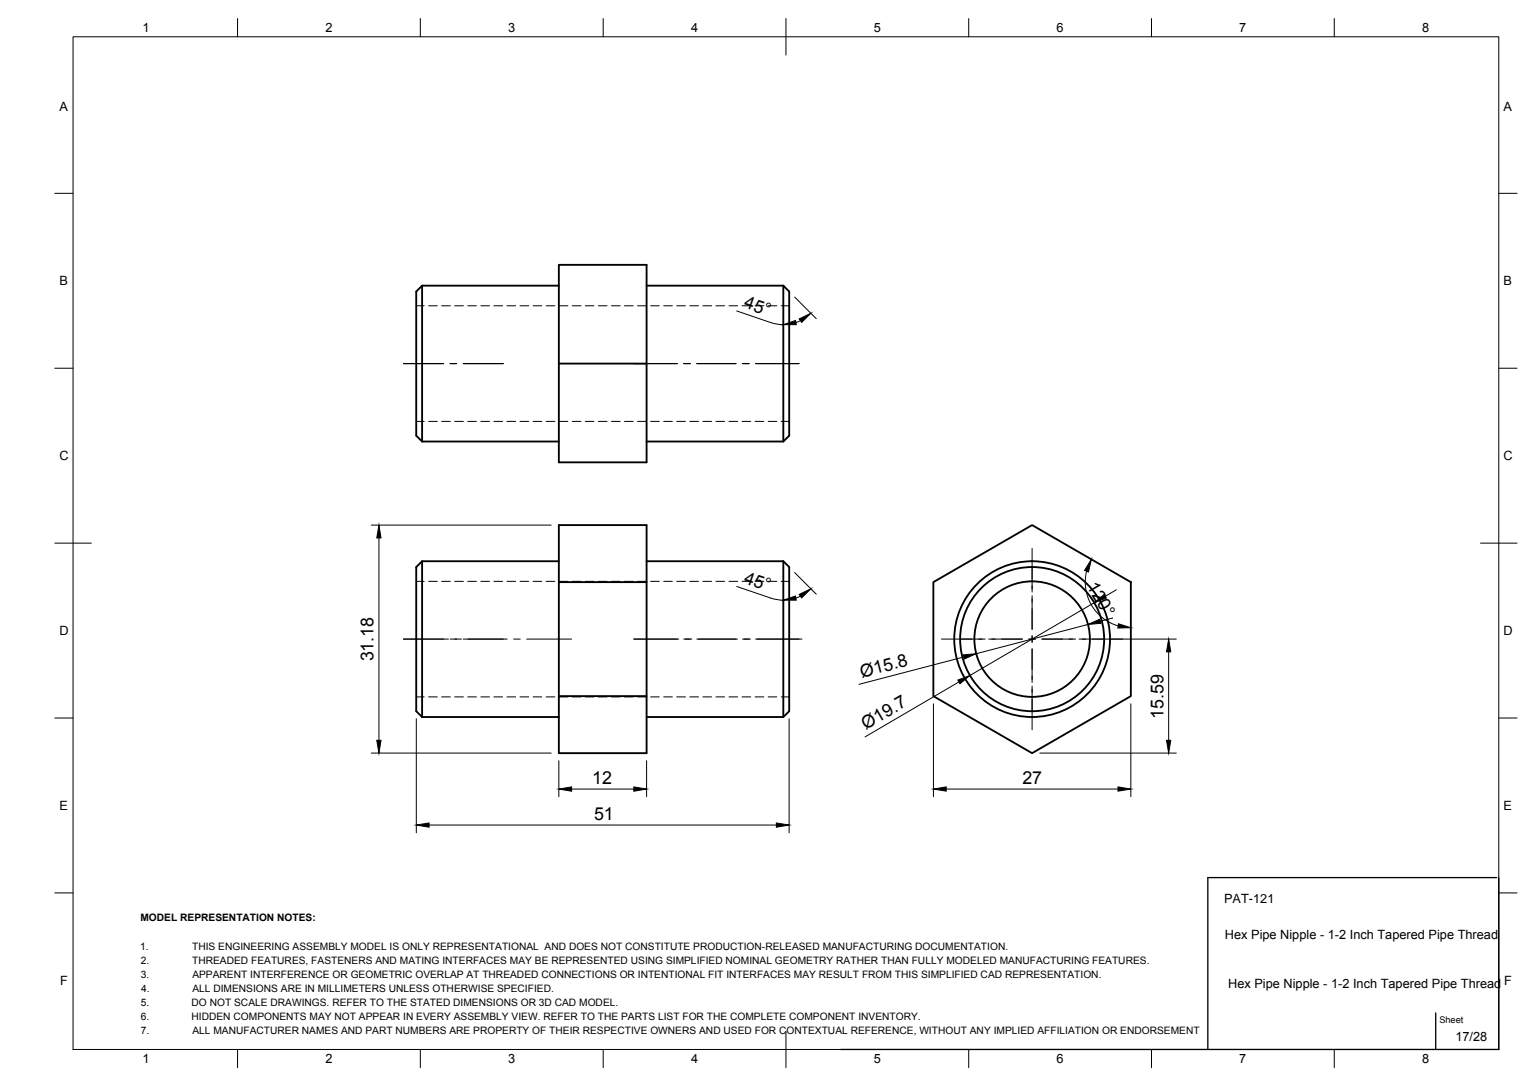
ISO-10303-21;
HEADER;
/* Generated by software containing ST-Developer
 * from STEP Tools, Inc. (www.steptools.com) 
 */

FILE_DESCRIPTION(
/* description */ ('Wall-mounted air drop station'),
/* implementation_level */ '2;1');

FILE_NAME(
/* name */ 'Hex Pipe Nipple - 1-2 Inch Tapered Pipe Thread.step',
/* time_stamp */ '2026-10-28T22:16:19-07:00',
/* author */ (''),
/* organization */ (''),
/* preprocessor_version */ 'ST-DEVELOPER v20.2',
/* originating_system */ 'Autodesk Translation Framework v15.17.0.0',
/* authorisation */ '');

FILE_SCHEMA (('AUTOMOTIVE_DESIGN { 1 0 10303 214 3 1 1 }'));
ENDSEC;

DATA;
#10=MECHANICAL_DESIGN_GEOMETRIC_PRESENTATION_REPRESENTATION('',(#360),#10517);
#273=CONICAL_SURFACE('',#6636,1.025,0.785398163397448);
#274=CONICAL_SURFACE('',#6639,1.025,0.785398163397448);
#302=SHAPE_REPRESENTATION_RELATIONSHIP('SRR','None',#10659,#331);
#331=ADVANCED_BREP_SHAPE_REPRESENTATION('',(#388),#10503);
#360=STYLED_ITEM('',(#10860),#388);
#388=MANIFOLD_SOLID_BREP('Body1',#5900);
#498=FACE_BOUND('',#1418,.T.);
#499=FACE_BOUND('',#1420,.T.);
#500=FACE_BOUND('',#1429,.T.);
#501=FACE_BOUND('',#1434,.T.);
#651=PLANE('',#6621);
#652=PLANE('',#6623);
#653=PLANE('',#6625);
#654=PLANE('',#6626);
#655=PLANE('',#6627);
#656=PLANE('',#6628);
#657=PLANE('',#6629);
#658=PLANE('',#6630);
#659=PLANE('',#6633);
#660=PLANE('',#6641);
#963=FACE_OUTER_BOUND('',#1417,.T.);
#964=FACE_OUTER_BOUND('',#1419,.T.);
#965=FACE_OUTER_BOUND('',#1421,.T.);
#966=FACE_OUTER_BOUND('',#1422,.T.);
#967=FACE_OUTER_BOUND('',#1423,.T.);
#968=FACE_OUTER_BOUND('',#1424,.T.);
#969=FACE_OUTER_BOUND('',#1425,.T.);
#970=FACE_OUTER_BOUND('',#1426,.T.);
#971=FACE_OUTER_BOUND('',#1427,.T.);
#972=FACE_OUTER_BOUND('',#1428,.T.);
#973=FACE_OUTER_BOUND('',#1430,.T.);
#974=FACE_OUTER_BOUND('',#1431,.T.);
#975=FACE_OUTER_BOUND('',#1432,.T.);
#976=FACE_OUTER_BOUND('',#1433,.T.);
#977=FACE_OUTER_BOUND('',#1435,.T.);
#1417=EDGE_LOOP('',(#4843,#4844,#4845,#4846,#4847,#4848));
#1418=EDGE_LOOP('',(#4849));
#1419=EDGE_LOOP('',(#4850,#4851,#4852,#4853,#4854,#4855));
#1420=EDGE_LOOP('',(#4856));
#1421=EDGE_LOOP('',(#4857,#4858,#4859,#4860));
#1422=EDGE_LOOP('',(#4861,#4862,#4863,#4864));
#1423=EDGE_LOOP('',(#4865,#4866,#4867,#4868));
#1424=EDGE_LOOP('',(#4869,#4870,#4871,#4872));
#1425=EDGE_LOOP('',(#4873,#4874,#4875,#4876));
#1426=EDGE_LOOP('',(#4877,#4878,#4879,#4880));
#1427=EDGE_LOOP('',(#4881,#4882,#4883,#4884));
#1428=EDGE_LOOP('',(#4885));
#1429=EDGE_LOOP('',(#4886));
#1430=EDGE_LOOP('',(#4887,#4888,#4889,#4890));
#1431=EDGE_LOOP('',(#4891,#4892,#4893,#4894));
#1432=EDGE_LOOP('',(#4895,#4896,#4897,#4898));
#1433=EDGE_LOOP('',(#4899));
#1434=EDGE_LOOP('',(#4900));
#1435=EDGE_LOOP('',(#4901,#4902,#4903,#4904));
#1856=LINE('',#9743,#2320);
#1857=LINE('',#9745,#2321);
#1858=LINE('',#9747,#2322);
#1859=LINE('',#9749,#2323);
#1860=LINE('',#9751,#2324);
#1861=LINE('',#9752,#2325);
#1862=LINE('',#9758,#2326);
#1863=LINE('',#9760,#2327);
#1864=LINE('',#9762,#2328);
#1865=LINE('',#9764,#2329);
#1866=LINE('',#9766,#2330);
#1867=LINE('',#9767,#2331);
#1868=LINE('',#9771,#2332);
#1869=LINE('',#9772,#2333);
#1870=LINE('',#9774,#2334);
#1871=LINE('',#9776,#2335);
#1872=LINE('',#9778,#2336);
#1873=LINE('',#9780,#2337);
#1874=LINE('',#9784,#2338);
#1875=LINE('',#9792,#2339);
#1876=LINE('',#9796,#2340);
#1877=LINE('',#9800,#2341);
#1878=LINE('',#9805,#2342);
#2320=VECTOR('',#7962,1.);
#2321=VECTOR('',#7963,1.);
#2322=VECTOR('',#7964,1.);
#2323=VECTOR('',#7965,1.);
#2324=VECTOR('',#7966,1.);
#2325=VECTOR('',#7967,1.);
#2326=VECTOR('',#7972,1.);
#2327=VECTOR('',#7973,1.);
#2328=VECTOR('',#7974,1.);
#2329=VECTOR('',#7975,1.);
#2330=VECTOR('',#7976,1.);
#2331=VECTOR('',#7977,1.);
#2332=VECTOR('',#7982,1.);
#2333=VECTOR('',#7983,1.);
#2334=VECTOR('',#7986,1.);
#2335=VECTOR('',#7989,1.);
#2336=VECTOR('',#7992,1.);
#2337=VECTOR('',#7995,1.);
#2338=VECTOR('',#8000,1.065);
#2339=VECTOR('',#8011,1.025);
#2340=VECTOR('',#8016,1.065);
#2341=VECTOR('',#8021,1.025);
#2342=VECTOR('',#8028,0.79);
#2679=CIRCLE('',#6622,1.065);
#2680=CIRCLE('',#6624,1.065);
#2681=CIRCLE('',#6632,1.065);
#2682=CIRCLE('',#6634,0.985);
#2683=CIRCLE('',#6635,0.79);
#2684=CIRCLE('',#6638,1.065);
#2685=CIRCLE('',#6640,0.985);
#2686=CIRCLE('',#6642,0.79);
#3053=VERTEX_POINT('',#9741);
#3054=VERTEX_POINT('',#9742);
#3055=VERTEX_POINT('',#9744);
#3056=VERTEX_POINT('',#9746);
#3057=VERTEX_POINT('',#9748);
#3058=VERTEX_POINT('',#9750);
#3059=VERTEX_POINT('',#9753);
#3060=VERTEX_POINT('',#9756);
#3061=VERTEX_POINT('',#9757);
#3062=VERTEX_POINT('',#9759);
#3063=VERTEX_POINT('',#9761);
#3064=VERTEX_POINT('',#9763);
#3065=VERTEX_POINT('',#9765);
#3066=VERTEX_POINT('',#9768);
#3067=VERTEX_POINT('',#9783);
#3068=VERTEX_POINT('',#9787);
#3069=VERTEX_POINT('',#9789);
#3070=VERTEX_POINT('',#9794);
#3071=VERTEX_POINT('',#9798);
#3072=VERTEX_POINT('',#9802);
#3679=EDGE_CURVE('',#3053,#3054,#1856,.T.);
#3680=EDGE_CURVE('',#3054,#3055,#1857,.T.);
#3681=EDGE_CURVE('',#3055,#3056,#1858,.T.);
#3682=EDGE_CURVE('',#3056,#3057,#1859,.T.);
#3683=EDGE_CURVE('',#3057,#3058,#1860,.T.);
#3684=EDGE_CURVE('',#3058,#3053,#1861,.T.);
#3685=EDGE_CURVE('',#3059,#3059,#2679,.T.);
#3686=EDGE_CURVE('',#3060,#3061,#1862,.T.);
#3687=EDGE_CURVE('',#3061,#3062,#1863,.T.);
#3688=EDGE_CURVE('',#3062,#3063,#1864,.T.);
#3689=EDGE_CURVE('',#3063,#3064,#1865,.T.);
#3690=EDGE_CURVE('',#3064,#3065,#1866,.T.);
#3691=EDGE_CURVE('',#3065,#3060,#1867,.T.);
#3692=EDGE_CURVE('',#3066,#3066,#2680,.T.);
#3693=EDGE_CURVE('',#3060,#3054,#1868,.T.);
#3694=EDGE_CURVE('',#3055,#3065,#1869,.T.);
#3695=EDGE_CURVE('',#3056,#3064,#1870,.T.);
#3696=EDGE_CURVE('',#3057,#3063,#1871,.T.);
#3697=EDGE_CURVE('',#3058,#3062,#1872,.T.);
#3698=EDGE_CURVE('',#3053,#3061,#1873,.T.);
#3699=EDGE_CURVE('',#3066,#3067,#1874,.T.);
#3700=EDGE_CURVE('',#3067,#3067,#2681,.T.);
#3701=EDGE_CURVE('',#3068,#3068,#2682,.T.);
#3702=EDGE_CURVE('',#3069,#3069,#2683,.T.);
#3703=EDGE_CURVE('',#3067,#3068,#1875,.T.);
#3704=EDGE_CURVE('',#3070,#3070,#2684,.T.);
#3705=EDGE_CURVE('',#3070,#3059,#1876,.T.);
#3706=EDGE_CURVE('',#3071,#3071,#2685,.T.);
#3707=EDGE_CURVE('',#3071,#3070,#1877,.T.);
#3708=EDGE_CURVE('',#3072,#3072,#2686,.T.);
#3709=EDGE_CURVE('',#3072,#3069,#1878,.T.);
#4843=ORIENTED_EDGE('',*,*,#3679,.T.);
#4844=ORIENTED_EDGE('',*,*,#3680,.T.);
#4845=ORIENTED_EDGE('',*,*,#3681,.T.);
#4846=ORIENTED_EDGE('',*,*,#3682,.T.);
#4847=ORIENTED_EDGE('',*,*,#3683,.T.);
#4848=ORIENTED_EDGE('',*,*,#3684,.T.);
#4849=ORIENTED_EDGE('',*,*,#3685,.F.);
#4850=ORIENTED_EDGE('',*,*,#3686,.T.);
#4851=ORIENTED_EDGE('',*,*,#3687,.T.);
#4852=ORIENTED_EDGE('',*,*,#3688,.T.);
#4853=ORIENTED_EDGE('',*,*,#3689,.T.);
#4854=ORIENTED_EDGE('',*,*,#3690,.T.);
#4855=ORIENTED_EDGE('',*,*,#3691,.T.);
#4856=ORIENTED_EDGE('',*,*,#3692,.F.);
#4857=ORIENTED_EDGE('',*,*,#3693,.F.);
#4858=ORIENTED_EDGE('',*,*,#3691,.F.);
#4859=ORIENTED_EDGE('',*,*,#3694,.F.);
#4860=ORIENTED_EDGE('',*,*,#3680,.F.);
#4861=ORIENTED_EDGE('',*,*,#3694,.T.);
#4862=ORIENTED_EDGE('',*,*,#3690,.F.);
#4863=ORIENTED_EDGE('',*,*,#3695,.F.);
#4864=ORIENTED_EDGE('',*,*,#3681,.F.);
#4865=ORIENTED_EDGE('',*,*,#3695,.T.);
#4866=ORIENTED_EDGE('',*,*,#3689,.F.);
#4867=ORIENTED_EDGE('',*,*,#3696,.F.);
#4868=ORIENTED_EDGE('',*,*,#3682,.F.);
#4869=ORIENTED_EDGE('',*,*,#3696,.T.);
#4870=ORIENTED_EDGE('',*,*,#3688,.F.);
#4871=ORIENTED_EDGE('',*,*,#3697,.F.);
#4872=ORIENTED_EDGE('',*,*,#3683,.F.);
#4873=ORIENTED_EDGE('',*,*,#3697,.T.);
#4874=ORIENTED_EDGE('',*,*,#3687,.F.);
#4875=ORIENTED_EDGE('',*,*,#3698,.F.);
#4876=ORIENTED_EDGE('',*,*,#3684,.F.);
#4877=ORIENTED_EDGE('',*,*,#3698,.T.);
#4878=ORIENTED_EDGE('',*,*,#3686,.F.);
#4879=ORIENTED_EDGE('',*,*,#3693,.T.);
#4880=ORIENTED_EDGE('',*,*,#3679,.F.);
#4881=ORIENTED_EDGE('',*,*,#3692,.T.);
#4882=ORIENTED_EDGE('',*,*,#3699,.T.);
#4883=ORIENTED_EDGE('',*,*,#3700,.T.);
#4884=ORIENTED_EDGE('',*,*,#3699,.F.);
#4885=ORIENTED_EDGE('',*,*,#3701,.F.);
#4886=ORIENTED_EDGE('',*,*,#3702,.T.);
#4887=ORIENTED_EDGE('',*,*,#3700,.F.);
#4888=ORIENTED_EDGE('',*,*,#3703,.T.);
#4889=ORIENTED_EDGE('',*,*,#3701,.T.);
#4890=ORIENTED_EDGE('',*,*,#3703,.F.);
#4891=ORIENTED_EDGE('',*,*,#3704,.F.);
#4892=ORIENTED_EDGE('',*,*,#3705,.T.);
#4893=ORIENTED_EDGE('',*,*,#3685,.T.);
#4894=ORIENTED_EDGE('',*,*,#3705,.F.);
#4895=ORIENTED_EDGE('',*,*,#3706,.F.);
#4896=ORIENTED_EDGE('',*,*,#3707,.T.);
#4897=ORIENTED_EDGE('',*,*,#3704,.T.);
#4898=ORIENTED_EDGE('',*,*,#3707,.F.);
#4899=ORIENTED_EDGE('',*,*,#3706,.T.);
#4900=ORIENTED_EDGE('',*,*,#3708,.F.);
#4901=ORIENTED_EDGE('',*,*,#3708,.T.);
#4902=ORIENTED_EDGE('',*,*,#3709,.T.);
#4903=ORIENTED_EDGE('',*,*,#3702,.F.);
#4904=ORIENTED_EDGE('',*,*,#3709,.F.);
#5501=CYLINDRICAL_SURFACE('',#6631,1.065);
#5502=CYLINDRICAL_SURFACE('',#6637,1.065);
#5503=CYLINDRICAL_SURFACE('',#6643,0.79);
#5736=ADVANCED_FACE('',(#963,#498),#651,.F.);
#5737=ADVANCED_FACE('',(#964,#499),#652,.T.);
#5738=ADVANCED_FACE('',(#965),#653,.T.);
#5739=ADVANCED_FACE('',(#966),#654,.T.);
#5740=ADVANCED_FACE('',(#967),#655,.T.);
#5741=ADVANCED_FACE('',(#968),#656,.T.);
#5742=ADVANCED_FACE('',(#969),#657,.T.);
#5743=ADVANCED_FACE('',(#970),#658,.T.);
#5744=ADVANCED_FACE('',(#971),#5501,.T.);
#5745=ADVANCED_FACE('',(#972,#500),#659,.T.);
#5746=ADVANCED_FACE('',(#973),#273,.T.);
#5747=ADVANCED_FACE('',(#974),#5502,.T.);
#5748=ADVANCED_FACE('',(#975),#274,.T.);
#5749=ADVANCED_FACE('',(#976,#501),#660,.T.);
#5750=ADVANCED_FACE('',(#977),#5503,.F.);
#5900=CLOSED_SHELL('',(#5736,#5737,#5738,#5739,#5740,#5741,#5742,#5743,
#5744,#5745,#5746,#5747,#5748,#5749,#5750));
#6620=AXIS2_PLACEMENT_3D('',#9739,#7958,#7959);
#6621=AXIS2_PLACEMENT_3D('',#9740,#7960,#7961);
#6622=AXIS2_PLACEMENT_3D('',#9754,#7968,#7969);
#6623=AXIS2_PLACEMENT_3D('',#9755,#7970,#7971);
#6624=AXIS2_PLACEMENT_3D('',#9769,#7978,#7979);
#6625=AXIS2_PLACEMENT_3D('',#9770,#7980,#7981);
#6626=AXIS2_PLACEMENT_3D('',#9773,#7984,#7985);
#6627=AXIS2_PLACEMENT_3D('',#9775,#7987,#7988);
#6628=AXIS2_PLACEMENT_3D('',#9777,#7990,#7991);
#6629=AXIS2_PLACEMENT_3D('',#9779,#7993,#7994);
#6630=AXIS2_PLACEMENT_3D('',#9781,#7996,#7997);
#6631=AXIS2_PLACEMENT_3D('',#9782,#7998,#7999);
#6632=AXIS2_PLACEMENT_3D('',#9785,#8001,#8002);
#6633=AXIS2_PLACEMENT_3D('',#9786,#8003,#8004);
#6634=AXIS2_PLACEMENT_3D('',#9788,#8005,#8006);
#6635=AXIS2_PLACEMENT_3D('',#9790,#8007,#8008);
#6636=AXIS2_PLACEMENT_3D('',#9791,#8009,#8010);
#6637=AXIS2_PLACEMENT_3D('',#9793,#8012,#8013);
#6638=AXIS2_PLACEMENT_3D('',#9795,#8014,#8015);
#6639=AXIS2_PLACEMENT_3D('',#9797,#8017,#8018);
#6640=AXIS2_PLACEMENT_3D('',#9799,#8019,#8020);
#6641=AXIS2_PLACEMENT_3D('',#9801,#8022,#8023);
#6642=AXIS2_PLACEMENT_3D('',#9803,#8024,#8025);
#6643=AXIS2_PLACEMENT_3D('',#9804,#8026,#8027);
#7958=DIRECTION('axis',(0.,0.,1.));
#7959=DIRECTION('refdir',(1.,0.,0.));
#7960=DIRECTION('center_axis',(0.,1.,0.));
#7961=DIRECTION('ref_axis',(1.,0.,0.));
#7962=DIRECTION('',(-0.5,0.,0.866025403784439));
#7963=DIRECTION('',(-1.,0.,-2.84883360945713E-16));
#7964=DIRECTION('',(-0.5,0.,-0.866025403784439));
#7965=DIRECTION('',(0.5,0.,-0.866025403784439));
#7966=DIRECTION('',(1.,0.,0.));
#7967=DIRECTION('',(0.5,0.,0.866025403784439));
#7968=DIRECTION('center_axis',(0.,-1.,0.));
#7969=DIRECTION('ref_axis',(1.,0.,0.));
#7970=DIRECTION('center_axis',(0.,1.,0.));
#7971=DIRECTION('ref_axis',(1.,0.,0.));
#7972=DIRECTION('',(0.5,0.,-0.866025403784439));
#7973=DIRECTION('',(-0.5,0.,-0.866025403784439));
#7974=DIRECTION('',(-1.,0.,0.));
#7975=DIRECTION('',(-0.5,0.,0.866025403784439));
#7976=DIRECTION('',(0.5,0.,0.866025403784439));
#7977=DIRECTION('',(1.,0.,2.84883360945713E-16));
#7978=DIRECTION('center_axis',(0.,1.,0.));
#7979=DIRECTION('ref_axis',(1.,0.,0.));
#7980=DIRECTION('center_axis',(-2.84883360945713E-16,0.,1.));
#7981=DIRECTION('ref_axis',(1.,0.,2.84883360945713E-16));
#7982=DIRECTION('',(0.,-1.,0.));
#7983=DIRECTION('',(0.,1.,0.));
#7984=DIRECTION('center_axis',(-0.866025403784439,0.,0.5));
#7985=DIRECTION('ref_axis',(0.5,0.,0.866025403784439));
#7986=DIRECTION('',(0.,1.,0.));
#7987=DIRECTION('center_axis',(-0.866025403784439,0.,-0.5));
#7988=DIRECTION('ref_axis',(-0.5,0.,0.866025403784439));
#7989=DIRECTION('',(0.,1.,0.));
#7990=DIRECTION('center_axis',(0.,0.,-1.));
#7991=DIRECTION('ref_axis',(-1.,0.,0.));
#7992=DIRECTION('',(0.,1.,0.));
#7993=DIRECTION('center_axis',(0.866025403784439,0.,-0.5));
#7994=DIRECTION('ref_axis',(-0.5,0.,-0.866025403784439));
#7995=DIRECTION('',(0.,1.,0.));
#7996=DIRECTION('center_axis',(0.866025403784439,0.,0.5));
#7997=DIRECTION('ref_axis',(0.5,0.,-0.866025403784439));
#7998=DIRECTION('center_axis',(0.,-1.,0.));
#7999=DIRECTION('ref_axis',(1.,0.,0.));
#8000=DIRECTION('',(0.,1.,0.));
#8001=DIRECTION('center_axis',(0.,-1.,0.));
#8002=DIRECTION('ref_axis',(1.,0.,0.));
#8003=DIRECTION('center_axis',(0.,1.,0.));
#8004=DIRECTION('ref_axis',(0.,0.,1.));
#8005=DIRECTION('center_axis',(0.,-1.,0.));
#8006=DIRECTION('ref_axis',(1.,0.,0.));
#8007=DIRECTION('center_axis',(0.,-1.,0.));
#8008=DIRECTION('ref_axis',(1.,0.,0.));
#8009=DIRECTION('center_axis',(0.,-1.,0.));
#8010=DIRECTION('ref_axis',(1.,0.,0.));
#8011=DIRECTION('',(0.707106781186547,0.707106781186548,8.65956056235493E-17));
#8012=DIRECTION('center_axis',(0.,-1.,0.));
#8013=DIRECTION('ref_axis',(1.,0.,0.));
#8014=DIRECTION('center_axis',(0.,-1.,0.));
#8015=DIRECTION('ref_axis',(1.,0.,0.));
#8016=DIRECTION('',(0.,1.,0.));
#8017=DIRECTION('center_axis',(0.,1.,0.));
#8018=DIRECTION('ref_axis',(1.,0.,0.));
#8019=DIRECTION('center_axis',(0.,-1.,0.));
#8020=DIRECTION('ref_axis',(1.,0.,0.));
#8021=DIRECTION('',(-0.707106781186547,0.707106781186548,-8.65956056235493E-17));
#8022=DIRECTION('center_axis',(0.,-1.,0.));
#8023=DIRECTION('ref_axis',(0.,0.,-1.));
#8024=DIRECTION('center_axis',(0.,-1.,0.));
#8025=DIRECTION('ref_axis',(1.,0.,0.));
#8026=DIRECTION('center_axis',(0.,-1.,0.));
#8027=DIRECTION('ref_axis',(1.,0.,0.));
#8028=DIRECTION('',(0.,1.,0.));
#9739=CARTESIAN_POINT('',(0.,0.,0.));
#9740=CARTESIAN_POINT('Origin',(0.,-0.6,0.));
#9741=CARTESIAN_POINT('',(1.55884572681199,-0.6,0.));
#9742=CARTESIAN_POINT('',(0.779422863405995,-0.6,1.35));
#9743=CARTESIAN_POINT('',(0.779422863405995,-0.6,1.35));
#9744=CARTESIAN_POINT('',(-0.779422863405996,-0.6,1.35));
#9745=CARTESIAN_POINT('',(-0.779422863405996,-0.6,1.35));
#9746=CARTESIAN_POINT('',(-1.55884572681199,-0.6,-1.90903542970483E-16));
#9747=CARTESIAN_POINT('',(-1.55884572681199,-0.6,-1.90903542970483E-16));
#9748=CARTESIAN_POINT('',(-0.779422863405995,-0.6,-1.35));
#9749=CARTESIAN_POINT('',(-0.779422863405995,-0.6,-1.35));
#9750=CARTESIAN_POINT('',(0.779422863405995,-0.6,-1.35));
#9751=CARTESIAN_POINT('',(0.779422863405995,-0.6,-1.35));
#9752=CARTESIAN_POINT('',(1.55884572681199,-0.6,0.));
#9753=CARTESIAN_POINT('',(-1.065,-0.6,-1.30424884109193E-16));
#9754=CARTESIAN_POINT('Origin',(0.,-0.6,0.));
#9755=CARTESIAN_POINT('Origin',(0.,0.6,0.));
#9756=CARTESIAN_POINT('',(0.779422863405995,0.6,1.35));
#9757=CARTESIAN_POINT('',(1.55884572681199,0.6,0.));
#9758=CARTESIAN_POINT('',(0.779422863405995,0.6,1.35));
#9759=CARTESIAN_POINT('',(0.779422863405995,0.6,-1.35));
#9760=CARTESIAN_POINT('',(1.55884572681199,0.6,0.));
#9761=CARTESIAN_POINT('',(-0.779422863405995,0.6,-1.35));
#9762=CARTESIAN_POINT('',(0.779422863405995,0.6,-1.35));
#9763=CARTESIAN_POINT('',(-1.55884572681199,0.6,-1.90903542970483E-16));
#9764=CARTESIAN_POINT('',(-0.779422863405995,0.6,-1.35));
#9765=CARTESIAN_POINT('',(-0.779422863405996,0.6,1.35));
#9766=CARTESIAN_POINT('',(-1.55884572681199,0.6,-1.90903542970483E-16));
#9767=CARTESIAN_POINT('',(-0.779422863405996,0.6,1.35));
#9768=CARTESIAN_POINT('',(-1.065,0.6,1.30424884109193E-16));
#9769=CARTESIAN_POINT('Origin',(0.,0.6,0.));
#9770=CARTESIAN_POINT('Origin',(-0.779422863405996,0.,1.35));
#9771=CARTESIAN_POINT('',(0.779422863405995,0.,1.35));
#9772=CARTESIAN_POINT('',(-0.779422863405996,0.,1.35));
#9773=CARTESIAN_POINT('Origin',(-1.55884572681199,0.,-1.90903542970483E-16));
#9774=CARTESIAN_POINT('',(-1.55884572681199,0.,-1.90903542970483E-16));
#9775=CARTESIAN_POINT('Origin',(-0.779422863405995,0.,-1.35));
#9776=CARTESIAN_POINT('',(-0.779422863405995,0.,-1.35));
#9777=CARTESIAN_POINT('Origin',(0.779422863405995,0.,-1.35));
#9778=CARTESIAN_POINT('',(0.779422863405995,0.,-1.35));
#9779=CARTESIAN_POINT('Origin',(1.55884572681199,0.,0.));
#9780=CARTESIAN_POINT('',(1.55884572681199,0.,0.));
#9781=CARTESIAN_POINT('Origin',(0.779422863405995,0.,1.35));
#9782=CARTESIAN_POINT('Origin',(0.,0.,0.));
#9783=CARTESIAN_POINT('',(-1.065,2.47,-1.30424884109193E-16));
#9784=CARTESIAN_POINT('',(-1.065,0.,-1.30424884109193E-16));
#9785=CARTESIAN_POINT('Origin',(0.,2.47,0.));
#9786=CARTESIAN_POINT('Origin',(0.985,2.55,0.));
#9787=CARTESIAN_POINT('',(-0.985,2.55,-1.20627709716014E-16));
#9788=CARTESIAN_POINT('Origin',(0.,2.55,0.));
#9789=CARTESIAN_POINT('',(-0.79,2.55,-9.67470971326409E-17));
#9790=CARTESIAN_POINT('Origin',(0.,2.55,0.));
#9791=CARTESIAN_POINT('Origin',(0.,2.51,0.));
#9792=CARTESIAN_POINT('',(-1.025,2.51,-1.25526296912604E-16));
#9793=CARTESIAN_POINT('Origin',(0.,0.,0.));
#9794=CARTESIAN_POINT('',(-1.065,-2.47,-1.30424884109193E-16));
#9795=CARTESIAN_POINT('Origin',(0.,-2.47,0.));
#9796=CARTESIAN_POINT('',(-1.065,0.,-1.30424884109193E-16));
#9797=CARTESIAN_POINT('Origin',(0.,-2.51,0.));
#9798=CARTESIAN_POINT('',(-0.985,-2.55,-1.20627709716014E-16));
#9799=CARTESIAN_POINT('Origin',(0.,-2.55,0.));
#9800=CARTESIAN_POINT('',(-1.025,-2.51,-1.25526296912604E-16));
#9801=CARTESIAN_POINT('Origin',(0.79,-2.55,0.));
#9802=CARTESIAN_POINT('',(-0.79,-2.55,-9.67470971326409E-17));
#9803=CARTESIAN_POINT('Origin',(0.,-2.55,0.));
#9804=CARTESIAN_POINT('Origin',(0.,0.,0.));
#9805=CARTESIAN_POINT('',(-0.79,0.,-9.67470971326409E-17));
#10470=UNCERTAINTY_MEASURE_WITH_UNIT(LENGTH_MEASURE(0.001),#10518,
'DISTANCE_ACCURACY_VALUE',
'Maximum model space distance between geometric entities at asserted c
onnectivities');
#10484=UNCERTAINTY_MEASURE_WITH_UNIT(LENGTH_MEASURE(0.001),#10518,
'DISTANCE_ACCURACY_VALUE',
'Maximum model space distance between geometric entities at asserted c
onnectivities');
#10503=(
GEOMETRIC_REPRESENTATION_CONTEXT(3)
GLOBAL_UNCERTAINTY_ASSIGNED_CONTEXT((#10470))
GLOBAL_UNIT_ASSIGNED_CONTEXT((#10518,#10520,#10521))
REPRESENTATION_CONTEXT('','3D')
);
#10517=(
GEOMETRIC_REPRESENTATION_CONTEXT(3)
GLOBAL_UNCERTAINTY_ASSIGNED_CONTEXT((#10484))
GLOBAL_UNIT_ASSIGNED_CONTEXT((#10518,#10520,#10521))
REPRESENTATION_CONTEXT('','3D')
);
#10518=(
LENGTH_UNIT()
NAMED_UNIT(*)
SI_UNIT(.CENTI.,.METRE.)
);
#10520=(
NAMED_UNIT(*)
PLANE_ANGLE_UNIT()
SI_UNIT($,.RADIAN.)
);
#10521=(
NAMED_UNIT(*)
SI_UNIT($,.STERADIAN.)
SOLID_ANGLE_UNIT()
);
#10540=SHAPE_DEFINITION_REPRESENTATION(#10572,#10659);
#10572=PRODUCT_DEFINITION_SHAPE('',$,#10692);
#10659=SHAPE_REPRESENTATION('',(#6620),#10503);
#10673=PRODUCT_DEFINITION_CONTEXT('part definition',#10771,'design');
#10692=PRODUCT_DEFINITION(
'Hex Pipe Nipple - 1-2 Inch Tapered Pipe Thread',
'Hex Pipe Nipple - 1-2 Inch Tapered Pipe Thread',#10724,#10673);
#10724=PRODUCT_DEFINITION_FORMATION('',$,#10791);
#10771=APPLICATION_CONTEXT(
'Core Data for Automotive Mechanical Design Process');
#10772=PRODUCT_CONTEXT('part definition',#10771,'mechanical');
#10791=PRODUCT('Hex Pipe Nipple - 1-2 Inch Tapered Pipe Thread',
'Hex Pipe Nipple - 1-2 Inch Tapered Pipe Thread',
'Hex Pipe Nipple - 1-2 Inch Tapered Pipe Thread',(#10772));
#10854=COLOUR_RGB('Light Blue',0.38,0.62,0.78);
#10855=FILL_AREA_STYLE_COLOUR('',#10854);
#10856=FILL_AREA_STYLE('',(#10855));
#10857=SURFACE_STYLE_FILL_AREA(#10856);
#10858=SURFACE_SIDE_STYLE('',(#10857));
#10859=SURFACE_STYLE_USAGE(.BOTH.,#10858);
#10860=PRESENTATION_STYLE_ASSIGNMENT((#10859));
ENDSEC;
END-ISO-10303-21;
